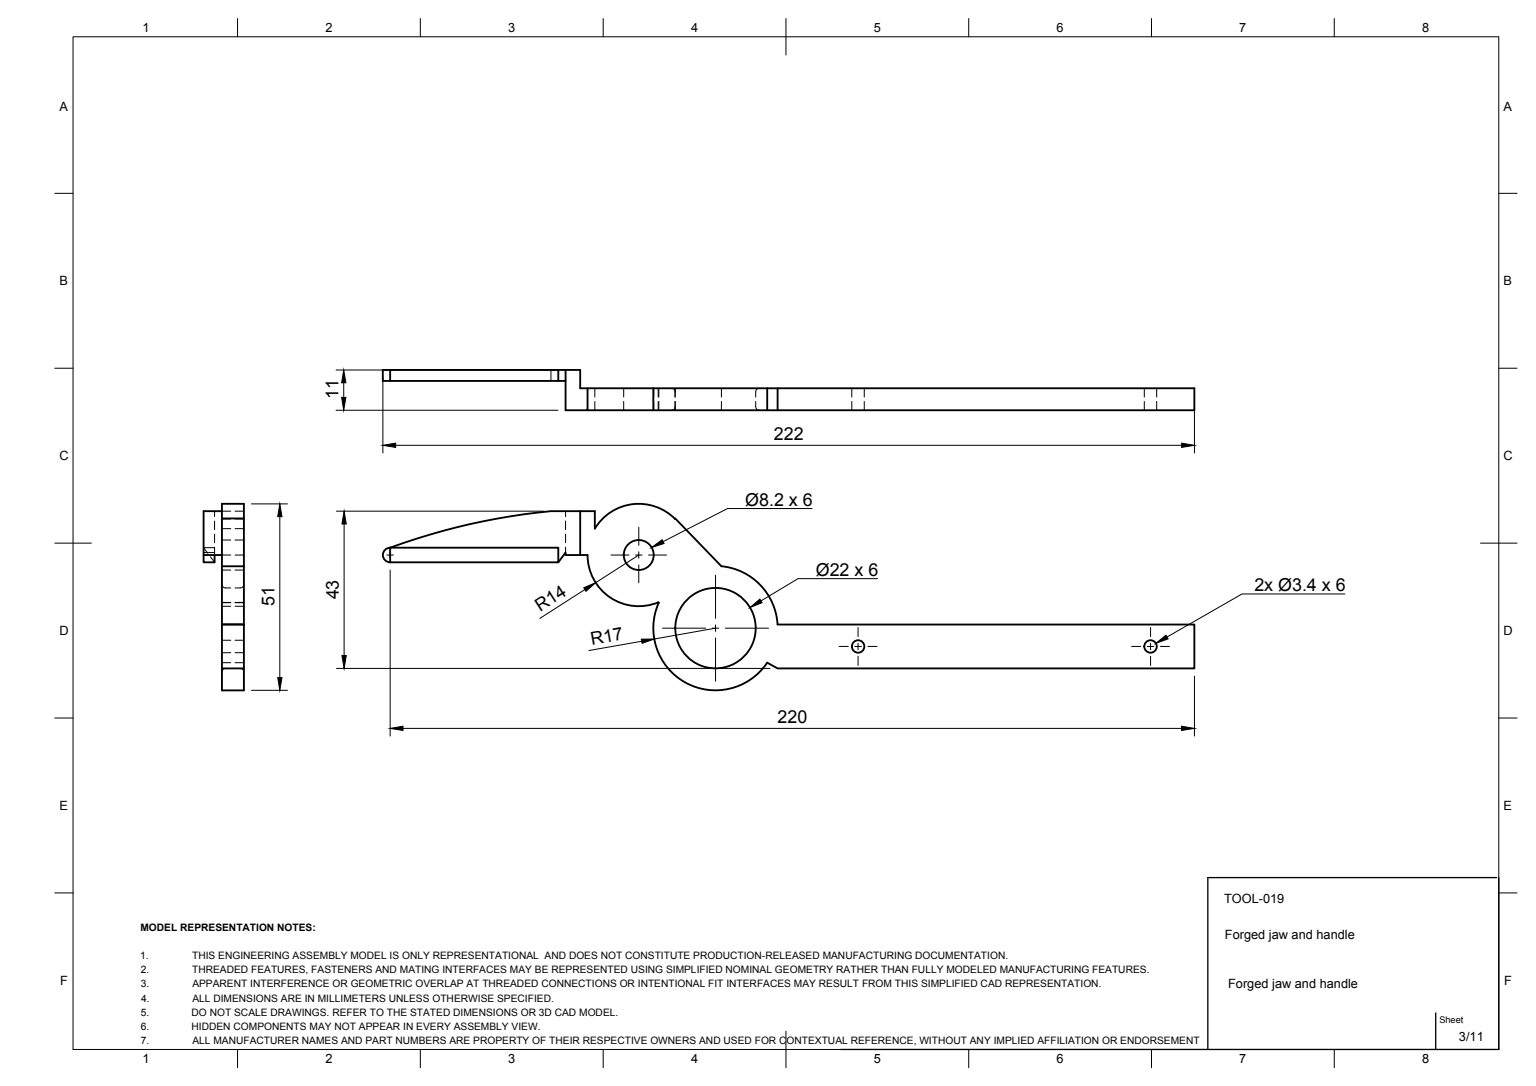
ISO-10303-21;
HEADER;
/* Generated by software containing ST-Developer
 * from STEP Tools, Inc. (www.steptools.com) 
 */

FILE_DESCRIPTION(
/* description */ (''),
/* implementation_level */ '2;1');

FILE_NAME(
/* name */ 'Forged jaw and handle.step',
/* time_stamp */ '2026-11-10T09:14:46-08:00',
/* author */ (''),
/* organization */ (''),
/* preprocessor_version */ 'ST-DEVELOPER v20.2',
/* originating_system */ 'Autodesk Translation Framework v15.17.0.0',
/* authorisation */ '');

FILE_SCHEMA (('AUTOMOTIVE_DESIGN { 1 0 10303 214 3 1 1 }'));
ENDSEC;

DATA;
#10=MECHANICAL_DESIGN_GEOMETRIC_PRESENTATION_REPRESENTATION('',(#558),#19471);
#538=SHAPE_REPRESENTATION_RELATIONSHIP('SRR','None',#19517,#548);
#548=ADVANCED_BREP_SHAPE_REPRESENTATION('',(#568),#19460);
#558=STYLED_ITEM('',(#19581),#568);
#568=MANIFOLD_SOLID_BREP('Body1',#7151);
#578=TOROIDAL_SURFACE('',#7315,1.2,0.1);
#579=TOROIDAL_SURFACE('',#7321,1.2,0.1);
#582=FACE_BOUND('',#1246,.T.);
#583=FACE_BOUND('',#1247,.T.);
#584=FACE_BOUND('',#1248,.T.);
#585=FACE_BOUND('',#1249,.T.);
#586=FACE_BOUND('',#1254,.T.);
#587=FACE_BOUND('',#1255,.T.);
#588=FACE_BOUND('',#1256,.T.);
#589=FACE_BOUND('',#1257,.T.);
#653=PLANE('',#7283);
#654=PLANE('',#7284);
#655=PLANE('',#7285);
#656=PLANE('',#7286);
#657=PLANE('',#7288);
#658=PLANE('',#7294);
#659=PLANE('',#7295);
#660=PLANE('',#7296);
#661=PLANE('',#7297);
#662=PLANE('',#7298);
#663=PLANE('',#7299);
#664=PLANE('',#7300);
#665=PLANE('',#7306);
#666=PLANE('',#7311);
#667=PLANE('',#7325);
#668=PLANE('',#7326);
#669=PLANE('',#7327);
#670=PLANE('',#7328);
#671=PLANE('',#7329);
#672=PLANE('',#7330);
#673=PLANE('',#7331);
#674=PLANE('',#7332);
#820=FACE_OUTER_BOUND('',#1229,.T.);
#821=FACE_OUTER_BOUND('',#1230,.T.);
#822=FACE_OUTER_BOUND('',#1231,.T.);
#823=FACE_OUTER_BOUND('',#1232,.T.);
#824=FACE_OUTER_BOUND('',#1233,.T.);
#825=FACE_OUTER_BOUND('',#1234,.T.);
#826=FACE_OUTER_BOUND('',#1235,.T.);
#827=FACE_OUTER_BOUND('',#1236,.T.);
#828=FACE_OUTER_BOUND('',#1237,.T.);
#829=FACE_OUTER_BOUND('',#1238,.T.);
#830=FACE_OUTER_BOUND('',#1239,.T.);
#831=FACE_OUTER_BOUND('',#1240,.T.);
#832=FACE_OUTER_BOUND('',#1241,.T.);
#833=FACE_OUTER_BOUND('',#1242,.T.);
#834=FACE_OUTER_BOUND('',#1243,.T.);
#835=FACE_OUTER_BOUND('',#1244,.T.);
#836=FACE_OUTER_BOUND('',#1245,.T.);
#837=FACE_OUTER_BOUND('',#1250,.T.);
#838=FACE_OUTER_BOUND('',#1251,.T.);
#839=FACE_OUTER_BOUND('',#1252,.T.);
#840=FACE_OUTER_BOUND('',#1253,.T.);
#841=FACE_OUTER_BOUND('',#1258,.T.);
#842=FACE_OUTER_BOUND('',#1259,.T.);
#843=FACE_OUTER_BOUND('',#1260,.T.);
#844=FACE_OUTER_BOUND('',#1261,.T.);
#845=FACE_OUTER_BOUND('',#1262,.T.);
#846=FACE_OUTER_BOUND('',#1263,.T.);
#847=FACE_OUTER_BOUND('',#1264,.T.);
#848=FACE_OUTER_BOUND('',#1265,.T.);
#849=FACE_OUTER_BOUND('',#1266,.T.);
#850=FACE_OUTER_BOUND('',#1267,.T.);
#851=FACE_OUTER_BOUND('',#1268,.T.);
#852=FACE_OUTER_BOUND('',#1269,.T.);
#853=FACE_OUTER_BOUND('',#1270,.T.);
#1229=EDGE_LOOP('',(#4541,#4542,#4543,#4544));
#1230=EDGE_LOOP('',(#4545,#4546,#4547,#4548));
#1231=EDGE_LOOP('',(#4549,#4550,#4551,#4552));
#1232=EDGE_LOOP('',(#4553,#4554,#4555));
#1233=EDGE_LOOP('',(#4556,#4557,#4558,#4559));
#1234=EDGE_LOOP('',(#4560,#4561,#4562));
#1235=EDGE_LOOP('',(#4563,#4564,#4565,#4566,#4567,#4568,#4569,#4570));
#1236=EDGE_LOOP('',(#4571,#4572,#4573,#4574));
#1237=EDGE_LOOP('',(#4575,#4576,#4577,#4578));
#1238=EDGE_LOOP('',(#4579,#4580,#4581,#4582));
#1239=EDGE_LOOP('',(#4583,#4584,#4585,#4586,#4587,#4588));
#1240=EDGE_LOOP('',(#4589,#4590,#4591,#4592,#4593,#4594));
#1241=EDGE_LOOP('',(#4595,#4596,#4597,#4598,#4599,#4600,#4601,#4602));
#1242=EDGE_LOOP('',(#4603,#4604,#4605,#4606));
#1243=EDGE_LOOP('',(#4607,#4608));
#1244=EDGE_LOOP('',(#4609,#4610,#4611,#4612,#4613,#4614));
#1245=EDGE_LOOP('',(#4615,#4616,#4617,#4618,#4619,#4620,#4621,#4622,#4623,
#4624,#4625,#4626,#4627,#4628,#4629,#4630));
#1246=EDGE_LOOP('',(#4631));
#1247=EDGE_LOOP('',(#4632));
#1248=EDGE_LOOP('',(#4633));
#1249=EDGE_LOOP('',(#4634));
#1250=EDGE_LOOP('',(#4635,#4636,#4637,#4638));
#1251=EDGE_LOOP('',(#4639,#4640,#4641,#4642));
#1252=EDGE_LOOP('',(#4643,#4644,#4645,#4646));
#1253=EDGE_LOOP('',(#4647,#4648,#4649,#4650,#4651,#4652,#4653,#4654,#4655,
#4656,#4657,#4658,#4659,#4660,#4661,#4662));
#1254=EDGE_LOOP('',(#4663));
#1255=EDGE_LOOP('',(#4664));
#1256=EDGE_LOOP('',(#4665));
#1257=EDGE_LOOP('',(#4666));
#1258=EDGE_LOOP('',(#4667,#4668,#4669,#4670));
#1259=EDGE_LOOP('',(#4671,#4672,#4673,#4674,#4675));
#1260=EDGE_LOOP('',(#4676,#4677,#4678,#4679,#4680));
#1261=EDGE_LOOP('',(#4681,#4682,#4683,#4684));
#1262=EDGE_LOOP('',(#4685,#4686,#4687,#4688));
#1263=EDGE_LOOP('',(#4689,#4690,#4691,#4692));
#1264=EDGE_LOOP('',(#4693,#4694,#4695,#4696));
#1265=EDGE_LOOP('',(#4697,#4698,#4699,#4700));
#1266=EDGE_LOOP('',(#4701,#4702,#4703,#4704));
#1267=EDGE_LOOP('',(#4705,#4706,#4707,#4708));
#1268=EDGE_LOOP('',(#4709,#4710,#4711,#4712));
#1269=EDGE_LOOP('',(#4713,#4714,#4715,#4716));
#1270=EDGE_LOOP('',(#4717,#4718,#4719,#4720));
#1709=LINE('',#9393,#2183);
#1710=LINE('',#9399,#2184);
#1711=LINE('',#9405,#2185);
#1712=LINE('',#9410,#2186);
#1713=LINE('',#9412,#2187);
#1714=LINE('',#9413,#2188);
#1715=LINE('',#9417,#2189);
#1716=LINE('',#9418,#2190);
#1717=LINE('',#9419,#2191);
#1718=LINE('',#9422,#2192);
#1719=LINE('',#9423,#2193);
#1720=LINE('',#9426,#2194);
#1721=LINE('',#9428,#2195);
#1722=LINE('',#9430,#2196);
#1723=LINE('',#9432,#2197);
#1724=LINE('',#9434,#2198);
#1725=LINE('',#9438,#2199);
#1726=LINE('',#9439,#2200);
#1727=LINE('',#9444,#2201);
#1728=LINE('',#9448,#2202);
#1729=LINE('',#9451,#2203);
#1730=LINE('',#9452,#2204);
#1731=LINE('',#9455,#2205);
#1732=LINE('',#9457,#2206);
#1733=LINE('',#9458,#2207);
#1734=LINE('',#9461,#2208);
#1735=LINE('',#9463,#2209);
#1736=LINE('',#9465,#2210);
#1737=LINE('',#9466,#2211);
#1738=LINE('',#9469,#2212);
#1739=LINE('',#9470,#2213);
#1740=LINE('',#9474,#2214);
#1741=LINE('',#9476,#2215);
#1742=LINE('',#9477,#2216);
#1743=LINE('',#9480,#2217);
#1744=LINE('',#9484,#2218);
#1745=LINE('',#9486,#2219);
#1746=LINE('',#9490,#2220);
#1747=LINE('',#9492,#2221);
#1748=LINE('',#9494,#2222);
#1749=LINE('',#9496,#2223);
#1750=LINE('',#9498,#2224);
#1751=LINE('',#9502,#2225);
#1752=LINE('',#9508,#2226);
#1753=LINE('',#9509,#2227);
#1754=LINE('',#9512,#2228);
#1755=LINE('',#9517,#2229);
#1756=LINE('',#9520,#2230);
#1757=LINE('',#9524,#2231);
#1758=LINE('',#9526,#2232);
#1759=LINE('',#9528,#2233);
#1760=LINE('',#9530,#2234);
#1761=LINE('',#9532,#2235);
#1762=LINE('',#9536,#2236);
#1763=LINE('',#9537,#2237);
#1764=LINE('',#9549,#2238);
#1765=LINE('',#9553,#2239);
#1766=LINE('',#9554,#2240);
#1767=LINE('',#9556,#2241);
#1768=LINE('',#9557,#2242);
#1769=LINE('',#9559,#2243);
#1770=LINE('',#9561,#2244);
#1771=LINE('',#9564,#2245);
#1772=LINE('',#9567,#2246);
#1773=LINE('',#9569,#2247);
#2183=VECTOR('',#7827,0.17);
#2184=VECTOR('',#7834,0.17);
#2185=VECTOR('',#7841,0.41);
#2186=VECTOR('',#7846,1.);
#2187=VECTOR('',#7847,1.);
#2188=VECTOR('',#7848,1.);
#2189=VECTOR('',#7851,1.);
#2190=VECTOR('',#7852,1.);
#2191=VECTOR('',#7853,1.);
#2192=VECTOR('',#7856,1.);
#2193=VECTOR('',#7857,1.);
#2194=VECTOR('',#7860,1.);
#2195=VECTOR('',#7861,1.);
#2196=VECTOR('',#7862,1.);
#2197=VECTOR('',#7863,1.);
#2198=VECTOR('',#7864,1.);
#2199=VECTOR('',#7869,1.);
#2200=VECTOR('',#7870,1.);
#2201=VECTOR('',#7877,1.);
#2202=VECTOR('',#7882,1.);
#2203=VECTOR('',#7885,1.);
#2204=VECTOR('',#7886,1.);
#2205=VECTOR('',#7889,1.);
#2206=VECTOR('',#7890,1.);
#2207=VECTOR('',#7891,1.);
#2208=VECTOR('',#7894,1.);
#2209=VECTOR('',#7895,1.);
#2210=VECTOR('',#7896,1.);
#2211=VECTOR('',#7897,1.);
#2212=VECTOR('',#7900,1.);
#2213=VECTOR('',#7901,1.);
#2214=VECTOR('',#7906,1.);
#2215=VECTOR('',#7907,1.);
#2216=VECTOR('',#7908,1.);
#2217=VECTOR('',#7911,1.);
#2218=VECTOR('',#7914,1.);
#2219=VECTOR('',#7915,1.);
#2220=VECTOR('',#7918,1.);
#2221=VECTOR('',#7919,1.);
#2222=VECTOR('',#7920,1.);
#2223=VECTOR('',#7921,1.);
#2224=VECTOR('',#7922,1.);
#2225=VECTOR('',#7925,1.);
#2226=VECTOR('',#7932,1.);
#2227=VECTOR('',#7933,1.);
#2228=VECTOR('',#7936,1.);
#2229=VECTOR('',#7943,1.);
#2230=VECTOR('',#7946,1.);
#2231=VECTOR('',#7949,1.);
#2232=VECTOR('',#7950,1.);
#2233=VECTOR('',#7951,1.);
#2234=VECTOR('',#7952,1.);
#2235=VECTOR('',#7953,1.);
#2236=VECTOR('',#7956,1.);
#2237=VECTOR('',#7957,1.);
#2238=VECTOR('',#7972,1.1);
#2239=VECTOR('',#7979,1.);
#2240=VECTOR('',#7980,1.);
#2241=VECTOR('',#7983,1.);
#2242=VECTOR('',#7984,1.);
#2243=VECTOR('',#7987,1.);
#2244=VECTOR('',#7990,1.);
#2245=VECTOR('',#7995,1.);
#2246=VECTOR('',#8000,1.);
#2247=VECTOR('',#8003,1.);
#2657=CIRCLE('',#7275,0.17);
#2658=CIRCLE('',#7276,0.17);
#2659=CIRCLE('',#7278,0.17);
#2660=CIRCLE('',#7279,0.17);
#2661=CIRCLE('',#7281,0.41);
#2662=CIRCLE('',#7282,0.41);
#2663=CIRCLE('',#7287,17.7082646568653);
#2664=CIRCLE('',#7290,0.2);
#2665=CIRCLE('',#7291,0.2);
#2666=CIRCLE('',#7293,17.7082646568653);
#2667=CIRCLE('',#7301,1.4);
#2668=CIRCLE('',#7302,1.7);
#2669=CIRCLE('',#7303,1.7);
#2670=CIRCLE('',#7304,1.4);
#2671=CIRCLE('',#7305,1.2);
#2672=CIRCLE('',#7308,1.4);
#2673=CIRCLE('',#7310,1.4);
#2674=CIRCLE('',#7312,1.7);
#2675=CIRCLE('',#7313,1.7);
#2676=CIRCLE('',#7314,1.2);
#2677=CIRCLE('',#7316,0.1);
#2678=CIRCLE('',#7317,1.1);
#2679=CIRCLE('',#7319,1.1);
#2680=CIRCLE('',#7320,1.1);
#2681=CIRCLE('',#7322,0.1);
#2847=VERTEX_POINT('',#9390);
#2848=VERTEX_POINT('',#9392);
#2849=VERTEX_POINT('',#9396);
#2850=VERTEX_POINT('',#9398);
#2851=VERTEX_POINT('',#9402);
#2852=VERTEX_POINT('',#9404);
#2853=VERTEX_POINT('',#9408);
#2854=VERTEX_POINT('',#9409);
#2855=VERTEX_POINT('',#9411);
#2856=VERTEX_POINT('',#9415);
#2857=VERTEX_POINT('',#9416);
#2858=VERTEX_POINT('',#9421);
#2859=VERTEX_POINT('',#9425);
#2860=VERTEX_POINT('',#9427);
#2861=VERTEX_POINT('',#9429);
#2862=VERTEX_POINT('',#9431);
#2863=VERTEX_POINT('',#9433);
#2864=VERTEX_POINT('',#9437);
#2865=VERTEX_POINT('',#9441);
#2866=VERTEX_POINT('',#9446);
#2867=VERTEX_POINT('',#9450);
#2868=VERTEX_POINT('',#9454);
#2869=VERTEX_POINT('',#9456);
#2870=VERTEX_POINT('',#9460);
#2871=VERTEX_POINT('',#9462);
#2872=VERTEX_POINT('',#9464);
#2873=VERTEX_POINT('',#9468);
#2874=VERTEX_POINT('',#9473);
#2875=VERTEX_POINT('',#9475);
#2876=VERTEX_POINT('',#9479);
#2877=VERTEX_POINT('',#9481);
#2878=VERTEX_POINT('',#9483);
#2879=VERTEX_POINT('',#9485);
#2880=VERTEX_POINT('',#9487);
#2881=VERTEX_POINT('',#9489);
#2882=VERTEX_POINT('',#9491);
#2883=VERTEX_POINT('',#9493);
#2884=VERTEX_POINT('',#9495);
#2885=VERTEX_POINT('',#9497);
#2886=VERTEX_POINT('',#9499);
#2887=VERTEX_POINT('',#9501);
#2888=VERTEX_POINT('',#9504);
#2889=VERTEX_POINT('',#9507);
#2890=VERTEX_POINT('',#9511);
#2891=VERTEX_POINT('',#9515);
#2892=VERTEX_POINT('',#9519);
#2893=VERTEX_POINT('',#9521);
#2894=VERTEX_POINT('',#9523);
#2895=VERTEX_POINT('',#9525);
#2896=VERTEX_POINT('',#9527);
#2897=VERTEX_POINT('',#9529);
#2898=VERTEX_POINT('',#9531);
#2899=VERTEX_POINT('',#9533);
#2900=VERTEX_POINT('',#9535);
#2901=VERTEX_POINT('',#9538);
#2902=VERTEX_POINT('',#9541);
#2903=VERTEX_POINT('',#9545);
#2904=VERTEX_POINT('',#9546);
#3511=EDGE_CURVE('',#2847,#2847,#2657,.T.);
#3512=EDGE_CURVE('',#2847,#2848,#1709,.T.);
#3513=EDGE_CURVE('',#2848,#2848,#2658,.T.);
#3514=EDGE_CURVE('',#2849,#2849,#2659,.T.);
#3515=EDGE_CURVE('',#2849,#2850,#1710,.T.);
#3516=EDGE_CURVE('',#2850,#2850,#2660,.T.);
#3517=EDGE_CURVE('',#2851,#2851,#2661,.T.);
#3518=EDGE_CURVE('',#2851,#2852,#1711,.T.);
#3519=EDGE_CURVE('',#2852,#2852,#2662,.T.);
#3520=EDGE_CURVE('',#2853,#2854,#1712,.T.);
#3521=EDGE_CURVE('',#2855,#2853,#1713,.T.);
#3522=EDGE_CURVE('',#2855,#2854,#1714,.T.);
#3523=EDGE_CURVE('',#2856,#2857,#1715,.T.);
#3524=EDGE_CURVE('',#2855,#2856,#1716,.T.);
#3525=EDGE_CURVE('',#2857,#2853,#1717,.T.);
#3526=EDGE_CURVE('',#2858,#2857,#1718,.T.);
#3527=EDGE_CURVE('',#2856,#2858,#1719,.T.);
#3528=EDGE_CURVE('',#2854,#2859,#1720,.T.);
#3529=EDGE_CURVE('',#2859,#2860,#1721,.T.);
#3530=EDGE_CURVE('',#2860,#2861,#1722,.T.);
#3531=EDGE_CURVE('',#2861,#2862,#1723,.T.);
#3532=EDGE_CURVE('',#2862,#2863,#1724,.T.);
#3533=EDGE_CURVE('',#2863,#2857,#2663,.T.);
#3534=EDGE_CURVE('',#2859,#2864,#1725,.T.);
#3535=EDGE_CURVE('',#2864,#2855,#1726,.T.);
#3536=EDGE_CURVE('',#2865,#2856,#2664,.T.);
#3537=EDGE_CURVE('',#2857,#2858,#2665,.T.);
#3538=EDGE_CURVE('',#2865,#2857,#1727,.T.);
#3539=EDGE_CURVE('',#2866,#2865,#2666,.T.);
#3540=EDGE_CURVE('',#2866,#2863,#1728,.T.);
#3541=EDGE_CURVE('',#2864,#2867,#1729,.T.);
#3542=EDGE_CURVE('',#2866,#2867,#1730,.T.);
#3543=EDGE_CURVE('',#2868,#2867,#1731,.T.);
#3544=EDGE_CURVE('',#2869,#2868,#1732,.T.);
#3545=EDGE_CURVE('',#2869,#2860,#1733,.T.);
#3546=EDGE_CURVE('',#2870,#2862,#1734,.T.);
#3547=EDGE_CURVE('',#2871,#2870,#1735,.T.);
#3548=EDGE_CURVE('',#2872,#2871,#1736,.T.);
#3549=EDGE_CURVE('',#2868,#2872,#1737,.T.);
#3550=EDGE_CURVE('',#2873,#2861,#1738,.T.);
#3551=EDGE_CURVE('',#2870,#2873,#1739,.T.);
#3552=EDGE_CURVE('',#2874,#2869,#1740,.T.);
#3553=EDGE_CURVE('',#2875,#2874,#1741,.T.);
#3554=EDGE_CURVE('',#2873,#2875,#1742,.T.);
#3555=EDGE_CURVE('',#2872,#2876,#1743,.T.);
#3556=EDGE_CURVE('',#2877,#2876,#2667,.T.);
#3557=EDGE_CURVE('',#2878,#2877,#1744,.T.);
#3558=EDGE_CURVE('',#2879,#2878,#1745,.T.);
#3559=EDGE_CURVE('',#2880,#2879,#2668,.T.);
#3560=EDGE_CURVE('',#2881,#2880,#1746,.T.);
#3561=EDGE_CURVE('',#2882,#2881,#1747,.T.);
#3562=EDGE_CURVE('',#2883,#2882,#1748,.T.);
#3563=EDGE_CURVE('',#2884,#2883,#1749,.T.);
#3564=EDGE_CURVE('',#2885,#2884,#1750,.T.);
#3565=EDGE_CURVE('',#2886,#2885,#2669,.T.);
#3566=EDGE_CURVE('',#2887,#2886,#1751,.T.);
#3567=EDGE_CURVE('',#2874,#2887,#2670,.T.);
#3568=EDGE_CURVE('',#2888,#2888,#2671,.T.);
#3569=EDGE_CURVE('',#2876,#2889,#1752,.T.);
#3570=EDGE_CURVE('',#2889,#2871,#1753,.T.);
#3571=EDGE_CURVE('',#2887,#2890,#1754,.T.);
#3572=EDGE_CURVE('',#2875,#2890,#2672,.T.);
#3573=EDGE_CURVE('',#2891,#2889,#2673,.T.);
#3574=EDGE_CURVE('',#2891,#2877,#1755,.T.);
#3575=EDGE_CURVE('',#2890,#2892,#1756,.T.);
#3576=EDGE_CURVE('',#2892,#2893,#2674,.T.);
#3577=EDGE_CURVE('',#2893,#2894,#1757,.T.);
#3578=EDGE_CURVE('',#2894,#2895,#1758,.T.);
#3579=EDGE_CURVE('',#2895,#2896,#1759,.T.);
#3580=EDGE_CURVE('',#2896,#2897,#1760,.T.);
#3581=EDGE_CURVE('',#2897,#2898,#1761,.T.);
#3582=EDGE_CURVE('',#2898,#2899,#2675,.T.);
#3583=EDGE_CURVE('',#2899,#2900,#1762,.T.);
#3584=EDGE_CURVE('',#2900,#2891,#1763,.T.);
#3585=EDGE_CURVE('',#2901,#2901,#2676,.T.);
#3586=EDGE_CURVE('',#2888,#2902,#2677,.T.);
#3587=EDGE_CURVE('',#2902,#2902,#2678,.T.);
#3588=EDGE_CURVE('',#2903,#2904,#2679,.T.);
#3589=EDGE_CURVE('',#2904,#2903,#2680,.T.);
#3590=EDGE_CURVE('',#2904,#2902,#1764,.T.);
#3591=EDGE_CURVE('',#2901,#2903,#2681,.T.);
#3592=EDGE_CURVE('',#2899,#2879,#1765,.T.);
#3593=EDGE_CURVE('',#2880,#2898,#1766,.T.);
#3594=EDGE_CURVE('',#2886,#2892,#1767,.T.);
#3595=EDGE_CURVE('',#2893,#2885,#1768,.T.);
#3596=EDGE_CURVE('',#2884,#2894,#1769,.T.);
#3597=EDGE_CURVE('',#2881,#2897,#1770,.T.);
#3598=EDGE_CURVE('',#2878,#2900,#1771,.T.);
#3599=EDGE_CURVE('',#2882,#2896,#1772,.T.);
#3600=EDGE_CURVE('',#2883,#2895,#1773,.T.);
#4541=ORIENTED_EDGE('',*,*,#3511,.F.);
#4542=ORIENTED_EDGE('',*,*,#3512,.T.);
#4543=ORIENTED_EDGE('',*,*,#3513,.F.);
#4544=ORIENTED_EDGE('',*,*,#3512,.F.);
#4545=ORIENTED_EDGE('',*,*,#3514,.F.);
#4546=ORIENTED_EDGE('',*,*,#3515,.T.);
#4547=ORIENTED_EDGE('',*,*,#3516,.F.);
#4548=ORIENTED_EDGE('',*,*,#3515,.F.);
#4549=ORIENTED_EDGE('',*,*,#3517,.F.);
#4550=ORIENTED_EDGE('',*,*,#3518,.T.);
#4551=ORIENTED_EDGE('',*,*,#3519,.F.);
#4552=ORIENTED_EDGE('',*,*,#3518,.F.);
#4553=ORIENTED_EDGE('',*,*,#3520,.F.);
#4554=ORIENTED_EDGE('',*,*,#3521,.F.);
#4555=ORIENTED_EDGE('',*,*,#3522,.T.);
#4556=ORIENTED_EDGE('',*,*,#3523,.F.);
#4557=ORIENTED_EDGE('',*,*,#3524,.F.);
#4558=ORIENTED_EDGE('',*,*,#3521,.T.);
#4559=ORIENTED_EDGE('',*,*,#3525,.F.);
#4560=ORIENTED_EDGE('',*,*,#3526,.F.);
#4561=ORIENTED_EDGE('',*,*,#3527,.F.);
#4562=ORIENTED_EDGE('',*,*,#3523,.T.);
#4563=ORIENTED_EDGE('',*,*,#3525,.T.);
#4564=ORIENTED_EDGE('',*,*,#3520,.T.);
#4565=ORIENTED_EDGE('',*,*,#3528,.T.);
#4566=ORIENTED_EDGE('',*,*,#3529,.T.);
#4567=ORIENTED_EDGE('',*,*,#3530,.T.);
#4568=ORIENTED_EDGE('',*,*,#3531,.T.);
#4569=ORIENTED_EDGE('',*,*,#3532,.T.);
#4570=ORIENTED_EDGE('',*,*,#3533,.T.);
#4571=ORIENTED_EDGE('',*,*,#3534,.F.);
#4572=ORIENTED_EDGE('',*,*,#3528,.F.);
#4573=ORIENTED_EDGE('',*,*,#3522,.F.);
#4574=ORIENTED_EDGE('',*,*,#3535,.F.);
#4575=ORIENTED_EDGE('',*,*,#3536,.T.);
#4576=ORIENTED_EDGE('',*,*,#3527,.T.);
#4577=ORIENTED_EDGE('',*,*,#3537,.F.);
#4578=ORIENTED_EDGE('',*,*,#3538,.F.);
#4579=ORIENTED_EDGE('',*,*,#3539,.T.);
#4580=ORIENTED_EDGE('',*,*,#3538,.T.);
#4581=ORIENTED_EDGE('',*,*,#3533,.F.);
#4582=ORIENTED_EDGE('',*,*,#3540,.F.);
#4583=ORIENTED_EDGE('',*,*,#3541,.F.);
#4584=ORIENTED_EDGE('',*,*,#3535,.T.);
#4585=ORIENTED_EDGE('',*,*,#3524,.T.);
#4586=ORIENTED_EDGE('',*,*,#3536,.F.);
#4587=ORIENTED_EDGE('',*,*,#3539,.F.);
#4588=ORIENTED_EDGE('',*,*,#3542,.T.);
#4589=ORIENTED_EDGE('',*,*,#3534,.T.);
#4590=ORIENTED_EDGE('',*,*,#3541,.T.);
#4591=ORIENTED_EDGE('',*,*,#3543,.F.);
#4592=ORIENTED_EDGE('',*,*,#3544,.F.);
#4593=ORIENTED_EDGE('',*,*,#3545,.T.);
#4594=ORIENTED_EDGE('',*,*,#3529,.F.);
#4595=ORIENTED_EDGE('',*,*,#3546,.F.);
#4596=ORIENTED_EDGE('',*,*,#3547,.F.);
#4597=ORIENTED_EDGE('',*,*,#3548,.F.);
#4598=ORIENTED_EDGE('',*,*,#3549,.F.);
#4599=ORIENTED_EDGE('',*,*,#3543,.T.);
#4600=ORIENTED_EDGE('',*,*,#3542,.F.);
#4601=ORIENTED_EDGE('',*,*,#3540,.T.);
#4602=ORIENTED_EDGE('',*,*,#3532,.F.);
#4603=ORIENTED_EDGE('',*,*,#3531,.F.);
#4604=ORIENTED_EDGE('',*,*,#3550,.F.);
#4605=ORIENTED_EDGE('',*,*,#3551,.F.);
#4606=ORIENTED_EDGE('',*,*,#3546,.T.);
#4607=ORIENTED_EDGE('',*,*,#3526,.T.);
#4608=ORIENTED_EDGE('',*,*,#3537,.T.);
#4609=ORIENTED_EDGE('',*,*,#3552,.F.);
#4610=ORIENTED_EDGE('',*,*,#3553,.F.);
#4611=ORIENTED_EDGE('',*,*,#3554,.F.);
#4612=ORIENTED_EDGE('',*,*,#3550,.T.);
#4613=ORIENTED_EDGE('',*,*,#3530,.F.);
#4614=ORIENTED_EDGE('',*,*,#3545,.F.);
#4615=ORIENTED_EDGE('',*,*,#3549,.T.);
#4616=ORIENTED_EDGE('',*,*,#3555,.T.);
#4617=ORIENTED_EDGE('',*,*,#3556,.F.);
#4618=ORIENTED_EDGE('',*,*,#3557,.F.);
#4619=ORIENTED_EDGE('',*,*,#3558,.F.);
#4620=ORIENTED_EDGE('',*,*,#3559,.F.);
#4621=ORIENTED_EDGE('',*,*,#3560,.F.);
#4622=ORIENTED_EDGE('',*,*,#3561,.F.);
#4623=ORIENTED_EDGE('',*,*,#3562,.F.);
#4624=ORIENTED_EDGE('',*,*,#3563,.F.);
#4625=ORIENTED_EDGE('',*,*,#3564,.F.);
#4626=ORIENTED_EDGE('',*,*,#3565,.F.);
#4627=ORIENTED_EDGE('',*,*,#3566,.F.);
#4628=ORIENTED_EDGE('',*,*,#3567,.F.);
#4629=ORIENTED_EDGE('',*,*,#3552,.T.);
#4630=ORIENTED_EDGE('',*,*,#3544,.T.);
#4631=ORIENTED_EDGE('',*,*,#3513,.T.);
#4632=ORIENTED_EDGE('',*,*,#3516,.T.);
#4633=ORIENTED_EDGE('',*,*,#3519,.T.);
#4634=ORIENTED_EDGE('',*,*,#3568,.F.);
#4635=ORIENTED_EDGE('',*,*,#3569,.F.);
#4636=ORIENTED_EDGE('',*,*,#3555,.F.);
#4637=ORIENTED_EDGE('',*,*,#3548,.T.);
#4638=ORIENTED_EDGE('',*,*,#3570,.F.);
#4639=ORIENTED_EDGE('',*,*,#3553,.T.);
#4640=ORIENTED_EDGE('',*,*,#3567,.T.);
#4641=ORIENTED_EDGE('',*,*,#3571,.T.);
#4642=ORIENTED_EDGE('',*,*,#3572,.F.);
#4643=ORIENTED_EDGE('',*,*,#3569,.T.);
#4644=ORIENTED_EDGE('',*,*,#3573,.F.);
#4645=ORIENTED_EDGE('',*,*,#3574,.T.);
#4646=ORIENTED_EDGE('',*,*,#3556,.T.);
#4647=ORIENTED_EDGE('',*,*,#3551,.T.);
#4648=ORIENTED_EDGE('',*,*,#3554,.T.);
#4649=ORIENTED_EDGE('',*,*,#3572,.T.);
#4650=ORIENTED_EDGE('',*,*,#3575,.T.);
#4651=ORIENTED_EDGE('',*,*,#3576,.T.);
#4652=ORIENTED_EDGE('',*,*,#3577,.T.);
#4653=ORIENTED_EDGE('',*,*,#3578,.T.);
#4654=ORIENTED_EDGE('',*,*,#3579,.T.);
#4655=ORIENTED_EDGE('',*,*,#3580,.T.);
#4656=ORIENTED_EDGE('',*,*,#3581,.T.);
#4657=ORIENTED_EDGE('',*,*,#3582,.T.);
#4658=ORIENTED_EDGE('',*,*,#3583,.T.);
#4659=ORIENTED_EDGE('',*,*,#3584,.T.);
#4660=ORIENTED_EDGE('',*,*,#3573,.T.);
#4661=ORIENTED_EDGE('',*,*,#3570,.T.);
#4662=ORIENTED_EDGE('',*,*,#3547,.T.);
#4663=ORIENTED_EDGE('',*,*,#3511,.T.);
#4664=ORIENTED_EDGE('',*,*,#3514,.T.);
#4665=ORIENTED_EDGE('',*,*,#3517,.T.);
#4666=ORIENTED_EDGE('',*,*,#3585,.F.);
#4667=ORIENTED_EDGE('',*,*,#3568,.T.);
#4668=ORIENTED_EDGE('',*,*,#3586,.T.);
#4669=ORIENTED_EDGE('',*,*,#3587,.T.);
#4670=ORIENTED_EDGE('',*,*,#3586,.F.);
#4671=ORIENTED_EDGE('',*,*,#3588,.F.);
#4672=ORIENTED_EDGE('',*,*,#3589,.F.);
#4673=ORIENTED_EDGE('',*,*,#3590,.T.);
#4674=ORIENTED_EDGE('',*,*,#3587,.F.);
#4675=ORIENTED_EDGE('',*,*,#3590,.F.);
#4676=ORIENTED_EDGE('',*,*,#3585,.T.);
#4677=ORIENTED_EDGE('',*,*,#3591,.T.);
#4678=ORIENTED_EDGE('',*,*,#3588,.T.);
#4679=ORIENTED_EDGE('',*,*,#3589,.T.);
#4680=ORIENTED_EDGE('',*,*,#3591,.F.);
#4681=ORIENTED_EDGE('',*,*,#3592,.F.);
#4682=ORIENTED_EDGE('',*,*,#3582,.F.);
#4683=ORIENTED_EDGE('',*,*,#3593,.F.);
#4684=ORIENTED_EDGE('',*,*,#3559,.T.);
#4685=ORIENTED_EDGE('',*,*,#3594,.F.);
#4686=ORIENTED_EDGE('',*,*,#3565,.T.);
#4687=ORIENTED_EDGE('',*,*,#3595,.F.);
#4688=ORIENTED_EDGE('',*,*,#3576,.F.);
#4689=ORIENTED_EDGE('',*,*,#3595,.T.);
#4690=ORIENTED_EDGE('',*,*,#3564,.T.);
#4691=ORIENTED_EDGE('',*,*,#3596,.T.);
#4692=ORIENTED_EDGE('',*,*,#3577,.F.);
#4693=ORIENTED_EDGE('',*,*,#3593,.T.);
#4694=ORIENTED_EDGE('',*,*,#3581,.F.);
#4695=ORIENTED_EDGE('',*,*,#3597,.F.);
#4696=ORIENTED_EDGE('',*,*,#3560,.T.);
#4697=ORIENTED_EDGE('',*,*,#3594,.T.);
#4698=ORIENTED_EDGE('',*,*,#3575,.F.);
#4699=ORIENTED_EDGE('',*,*,#3571,.F.);
#4700=ORIENTED_EDGE('',*,*,#3566,.T.);
#4701=ORIENTED_EDGE('',*,*,#3574,.F.);
#4702=ORIENTED_EDGE('',*,*,#3584,.F.);
#4703=ORIENTED_EDGE('',*,*,#3598,.F.);
#4704=ORIENTED_EDGE('',*,*,#3557,.T.);
#4705=ORIENTED_EDGE('',*,*,#3592,.T.);
#4706=ORIENTED_EDGE('',*,*,#3558,.T.);
#4707=ORIENTED_EDGE('',*,*,#3598,.T.);
#4708=ORIENTED_EDGE('',*,*,#3583,.F.);
#4709=ORIENTED_EDGE('',*,*,#3561,.T.);
#4710=ORIENTED_EDGE('',*,*,#3597,.T.);
#4711=ORIENTED_EDGE('',*,*,#3580,.F.);
#4712=ORIENTED_EDGE('',*,*,#3599,.F.);
#4713=ORIENTED_EDGE('',*,*,#3562,.T.);
#4714=ORIENTED_EDGE('',*,*,#3599,.T.);
#4715=ORIENTED_EDGE('',*,*,#3579,.F.);
#4716=ORIENTED_EDGE('',*,*,#3600,.F.);
#4717=ORIENTED_EDGE('',*,*,#3563,.T.);
#4718=ORIENTED_EDGE('',*,*,#3600,.T.);
#4719=ORIENTED_EDGE('',*,*,#3578,.F.);
#4720=ORIENTED_EDGE('',*,*,#3596,.F.);
#6601=CYLINDRICAL_SURFACE('',#7274,0.17);
#6602=CYLINDRICAL_SURFACE('',#7277,0.17);
#6603=CYLINDRICAL_SURFACE('',#7280,0.41);
#6604=CYLINDRICAL_SURFACE('',#7289,0.2);
#6605=CYLINDRICAL_SURFACE('',#7292,17.7082646568653);
#6606=CYLINDRICAL_SURFACE('',#7307,1.4);
#6607=CYLINDRICAL_SURFACE('',#7309,1.4);
#6608=CYLINDRICAL_SURFACE('',#7318,1.1);
#6609=CYLINDRICAL_SURFACE('',#7323,1.7);
#6610=CYLINDRICAL_SURFACE('',#7324,1.7);
#6742=ADVANCED_FACE('',(#820),#6601,.F.);
#6743=ADVANCED_FACE('',(#821),#6602,.F.);
#6744=ADVANCED_FACE('',(#822),#6603,.F.);
#6745=ADVANCED_FACE('',(#823),#653,.F.);
#6746=ADVANCED_FACE('',(#824),#654,.F.);
#6747=ADVANCED_FACE('',(#825),#655,.T.);
#6748=ADVANCED_FACE('',(#826),#656,.T.);
#6749=ADVANCED_FACE('',(#827),#657,.T.);
#6750=ADVANCED_FACE('',(#828),#6604,.T.);
#6751=ADVANCED_FACE('',(#829),#6605,.T.);
#6752=ADVANCED_FACE('',(#830),#658,.F.);
#6753=ADVANCED_FACE('',(#831),#659,.T.);
#6754=ADVANCED_FACE('',(#832),#660,.T.);
#6755=ADVANCED_FACE('',(#833),#661,.T.);
#6756=ADVANCED_FACE('',(#834),#662,.T.);
#6757=ADVANCED_FACE('',(#835),#663,.T.);
#6758=ADVANCED_FACE('',(#836,#582,#583,#584,#585),#664,.F.);
#6759=ADVANCED_FACE('',(#837),#665,.T.);
#6760=ADVANCED_FACE('',(#838),#6606,.T.);
#6761=ADVANCED_FACE('',(#839),#6607,.T.);
#6762=ADVANCED_FACE('',(#840,#586,#587,#588,#589),#666,.T.);
#6763=ADVANCED_FACE('',(#841),#578,.T.);
#6764=ADVANCED_FACE('',(#842),#6608,.F.);
#6765=ADVANCED_FACE('',(#843),#579,.T.);
#6766=ADVANCED_FACE('',(#844),#6609,.T.);
#6767=ADVANCED_FACE('',(#845),#6610,.T.);
#6768=ADVANCED_FACE('',(#846),#667,.T.);
#6769=ADVANCED_FACE('',(#847),#668,.T.);
#6770=ADVANCED_FACE('',(#848),#669,.T.);
#6771=ADVANCED_FACE('',(#849),#670,.T.);
#6772=ADVANCED_FACE('',(#850),#671,.T.);
#6773=ADVANCED_FACE('',(#851),#672,.T.);
#6774=ADVANCED_FACE('',(#852),#673,.T.);
#6775=ADVANCED_FACE('',(#853),#674,.T.);
#7151=CLOSED_SHELL('',(#6742,#6743,#6744,#6745,#6746,#6747,#6748,#6749,
#6750,#6751,#6752,#6753,#6754,#6755,#6756,#6757,#6758,#6759,#6760,#6761,
#6762,#6763,#6764,#6765,#6766,#6767,#6768,#6769,#6770,#6771,#6772,#6773,
#6774,#6775));
#7273=AXIS2_PLACEMENT_3D('',#9388,#7821,#7822);
#7274=AXIS2_PLACEMENT_3D('',#9389,#7823,#7824);
#7275=AXIS2_PLACEMENT_3D('',#9391,#7825,#7826);
#7276=AXIS2_PLACEMENT_3D('',#9394,#7828,#7829);
#7277=AXIS2_PLACEMENT_3D('',#9395,#7830,#7831);
#7278=AXIS2_PLACEMENT_3D('',#9397,#7832,#7833);
#7279=AXIS2_PLACEMENT_3D('',#9400,#7835,#7836);
#7280=AXIS2_PLACEMENT_3D('',#9401,#7837,#7838);
#7281=AXIS2_PLACEMENT_3D('',#9403,#7839,#7840);
#7282=AXIS2_PLACEMENT_3D('',#9406,#7842,#7843);
#7283=AXIS2_PLACEMENT_3D('',#9407,#7844,#7845);
#7284=AXIS2_PLACEMENT_3D('',#9414,#7849,#7850);
#7285=AXIS2_PLACEMENT_3D('',#9420,#7854,#7855);
#7286=AXIS2_PLACEMENT_3D('',#9424,#7858,#7859);
#7287=AXIS2_PLACEMENT_3D('',#9435,#7865,#7866);
#7288=AXIS2_PLACEMENT_3D('',#9436,#7867,#7868);
#7289=AXIS2_PLACEMENT_3D('',#9440,#7871,#7872);
#7290=AXIS2_PLACEMENT_3D('',#9442,#7873,#7874);
#7291=AXIS2_PLACEMENT_3D('',#9443,#7875,#7876);
#7292=AXIS2_PLACEMENT_3D('',#9445,#7878,#7879);
#7293=AXIS2_PLACEMENT_3D('',#9447,#7880,#7881);
#7294=AXIS2_PLACEMENT_3D('',#9449,#7883,#7884);
#7295=AXIS2_PLACEMENT_3D('',#9453,#7887,#7888);
#7296=AXIS2_PLACEMENT_3D('',#9459,#7892,#7893);
#7297=AXIS2_PLACEMENT_3D('',#9467,#7898,#7899);
#7298=AXIS2_PLACEMENT_3D('',#9471,#7902,#7903);
#7299=AXIS2_PLACEMENT_3D('',#9472,#7904,#7905);
#7300=AXIS2_PLACEMENT_3D('',#9478,#7909,#7910);
#7301=AXIS2_PLACEMENT_3D('',#9482,#7912,#7913);
#7302=AXIS2_PLACEMENT_3D('',#9488,#7916,#7917);
#7303=AXIS2_PLACEMENT_3D('',#9500,#7923,#7924);
#7304=AXIS2_PLACEMENT_3D('',#9503,#7926,#7927);
#7305=AXIS2_PLACEMENT_3D('',#9505,#7928,#7929);
#7306=AXIS2_PLACEMENT_3D('',#9506,#7930,#7931);
#7307=AXIS2_PLACEMENT_3D('',#9510,#7934,#7935);
#7308=AXIS2_PLACEMENT_3D('',#9513,#7937,#7938);
#7309=AXIS2_PLACEMENT_3D('',#9514,#7939,#7940);
#7310=AXIS2_PLACEMENT_3D('',#9516,#7941,#7942);
#7311=AXIS2_PLACEMENT_3D('',#9518,#7944,#7945);
#7312=AXIS2_PLACEMENT_3D('',#9522,#7947,#7948);
#7313=AXIS2_PLACEMENT_3D('',#9534,#7954,#7955);
#7314=AXIS2_PLACEMENT_3D('',#9539,#7958,#7959);
#7315=AXIS2_PLACEMENT_3D('',#9540,#7960,#7961);
#7316=AXIS2_PLACEMENT_3D('',#9542,#7962,#7963);
#7317=AXIS2_PLACEMENT_3D('',#9543,#7964,#7965);
#7318=AXIS2_PLACEMENT_3D('',#9544,#7966,#7967);
#7319=AXIS2_PLACEMENT_3D('',#9547,#7968,#7969);
#7320=AXIS2_PLACEMENT_3D('',#9548,#7970,#7971);
#7321=AXIS2_PLACEMENT_3D('',#9550,#7973,#7974);
#7322=AXIS2_PLACEMENT_3D('',#9551,#7975,#7976);
#7323=AXIS2_PLACEMENT_3D('',#9552,#7977,#7978);
#7324=AXIS2_PLACEMENT_3D('',#9555,#7981,#7982);
#7325=AXIS2_PLACEMENT_3D('',#9558,#7985,#7986);
#7326=AXIS2_PLACEMENT_3D('',#9560,#7988,#7989);
#7327=AXIS2_PLACEMENT_3D('',#9562,#7991,#7992);
#7328=AXIS2_PLACEMENT_3D('',#9563,#7993,#7994);
#7329=AXIS2_PLACEMENT_3D('',#9565,#7996,#7997);
#7330=AXIS2_PLACEMENT_3D('',#9566,#7998,#7999);
#7331=AXIS2_PLACEMENT_3D('',#9568,#8001,#8002);
#7332=AXIS2_PLACEMENT_3D('',#9570,#8004,#8005);
#7821=DIRECTION('axis',(0.,0.,1.));
#7822=DIRECTION('refdir',(1.,0.,0.));
#7823=DIRECTION('center_axis',(0.,0.,-1.));
#7824=DIRECTION('ref_axis',(1.,0.,0.));
#7825=DIRECTION('center_axis',(0.,0.,-1.));
#7826=DIRECTION('ref_axis',(1.,0.,0.));
#7827=DIRECTION('',(0.,0.,-1.));
#7828=DIRECTION('center_axis',(0.,0.,1.));
#7829=DIRECTION('ref_axis',(1.,0.,0.));
#7830=DIRECTION('center_axis',(0.,0.,-1.));
#7831=DIRECTION('ref_axis',(1.,0.,0.));
#7832=DIRECTION('center_axis',(0.,0.,-1.));
#7833=DIRECTION('ref_axis',(1.,0.,0.));
#7834=DIRECTION('',(0.,0.,-1.));
#7835=DIRECTION('center_axis',(0.,0.,1.));
#7836=DIRECTION('ref_axis',(1.,0.,0.));
#7837=DIRECTION('center_axis',(0.,0.,-1.));
#7838=DIRECTION('ref_axis',(1.,0.,0.));
#7839=DIRECTION('center_axis',(0.,0.,-1.));
#7840=DIRECTION('ref_axis',(1.,0.,0.));
#7841=DIRECTION('',(0.,0.,-1.));
#7842=DIRECTION('center_axis',(0.,0.,1.));
#7843=DIRECTION('ref_axis',(1.,0.,0.));
#7844=DIRECTION('center_axis',(1.,0.,0.));
#7845=DIRECTION('ref_axis',(0.,0.,-1.));
#7846=DIRECTION('',(0.,-1.,0.));
#7847=DIRECTION('',(0.,0.8,0.6));
#7848=DIRECTION('',(0.,0.,1.));
#7849=DIRECTION('center_axis',(0.,0.6,-0.8));
#7850=DIRECTION('ref_axis',(0.,0.8,0.6));
#7851=DIRECTION('',(0.,0.8,0.6));
#7852=DIRECTION('',(-1.,0.,0.));
#7853=DIRECTION('',(1.,0.,0.));
#7854=DIRECTION('center_axis',(1.,0.,0.));
#7855=DIRECTION('ref_axis',(0.,2.22044604925031E-16,1.));
#7856=DIRECTION('',(0.,1.,0.));
#7857=DIRECTION('',(0.,0.,1.));
#7858=DIRECTION('center_axis',(0.,0.,1.));
#7859=DIRECTION('ref_axis',(1.,0.,0.));
#7860=DIRECTION('',(0.6,0.8,0.));
#7861=DIRECTION('',(0.,-1.,0.));
#7862=DIRECTION('',(1.,0.,0.));
#7863=DIRECTION('',(0.,1.,0.));
#7864=DIRECTION('',(-1.,0.,0.));
#7865=DIRECTION('center_axis',(0.,0.,1.));
#7866=DIRECTION('ref_axis',(-0.0955793180441842,0.995421817101779,0.));
#7867=DIRECTION('center_axis',(0.8,-0.6,0.));
#7868=DIRECTION('ref_axis',(0.6,0.8,0.));
#7869=DIRECTION('',(0.,0.,-1.));
#7870=DIRECTION('',(-0.6,-0.8,0.));
#7871=DIRECTION('center_axis',(0.,0.,1.));
#7872=DIRECTION('ref_axis',(4.44089209850063E-15,1.,0.));
#7873=DIRECTION('center_axis',(0.,0.,1.));
#7874=DIRECTION('ref_axis',(4.44089209850063E-15,1.,0.));
#7875=DIRECTION('center_axis',(0.,0.,1.));
#7876=DIRECTION('ref_axis',(4.44089209850063E-15,1.,0.));
#7877=DIRECTION('',(0.,0.,1.));
#7878=DIRECTION('center_axis',(0.,0.,1.));
#7879=DIRECTION('ref_axis',(-0.0955793180441842,0.995421817101779,0.));
#7880=DIRECTION('center_axis',(0.,0.,1.));
#7881=DIRECTION('ref_axis',(-0.0955793180441842,0.995421817101779,0.));
#7882=DIRECTION('',(0.,0.,1.));
#7883=DIRECTION('center_axis',(0.,0.,1.));
#7884=DIRECTION('ref_axis',(1.,0.,0.));
#7885=DIRECTION('',(0.,1.,0.));
#7886=DIRECTION('',(1.,0.,0.));
#7887=DIRECTION('center_axis',(-1.,0.,0.));
#7888=DIRECTION('ref_axis',(0.,-1.,0.));
#7889=DIRECTION('',(0.,0.,1.));
#7890=DIRECTION('',(0.,1.,0.));
#7891=DIRECTION('',(0.,0.,1.));
#7892=DIRECTION('center_axis',(0.,1.,0.));
#7893=DIRECTION('ref_axis',(-1.,0.,0.));
#7894=DIRECTION('',(0.,0.,1.));
#7895=DIRECTION('',(-1.,0.,0.));
#7896=DIRECTION('',(0.,0.,1.));
#7897=DIRECTION('',(1.,0.,0.));
#7898=DIRECTION('center_axis',(1.,0.,0.));
#7899=DIRECTION('ref_axis',(0.,1.,0.));
#7900=DIRECTION('',(0.,0.,1.));
#7901=DIRECTION('',(0.,-1.,0.));
#7902=DIRECTION('center_axis',(0.,0.,1.));
#7903=DIRECTION('ref_axis',(1.,0.,0.));
#7904=DIRECTION('center_axis',(0.,-1.,0.));
#7905=DIRECTION('ref_axis',(1.,0.,0.));
#7906=DIRECTION('',(-1.,0.,0.));
#7907=DIRECTION('',(0.,0.,-1.));
#7908=DIRECTION('',(1.,0.,0.));
#7909=DIRECTION('center_axis',(0.,0.,1.));
#7910=DIRECTION('ref_axis',(1.,0.,0.));
#7911=DIRECTION('',(0.,-1.,0.));
#7912=DIRECTION('center_axis',(0.,0.,1.));
#7913=DIRECTION('ref_axis',(1.,0.,0.));
#7914=DIRECTION('',(-0.447213595499958,-0.894427190999916,0.));
#7915=DIRECTION('',(-0.694594513699567,0.719401460617409,0.));
#7916=DIRECTION('center_axis',(0.,0.,1.));
#7917=DIRECTION('ref_axis',(1.,0.,0.));
#7918=DIRECTION('',(-0.694594513699567,0.719401460617409,0.));
#7919=DIRECTION('',(-1.,0.,0.));
#7920=DIRECTION('',(0.,1.,0.));
#7921=DIRECTION('',(1.,0.,0.));
#7922=DIRECTION('',(0.87524153543927,-0.483686111690123,0.));
#7923=DIRECTION('center_axis',(0.,0.,1.));
#7924=DIRECTION('ref_axis',(1.,0.,0.));
#7925=DIRECTION('',(0.87524153543927,-0.483686111690123,0.));
#7926=DIRECTION('center_axis',(0.,0.,1.));
#7927=DIRECTION('ref_axis',(1.,0.,0.));
#7928=DIRECTION('center_axis',(0.,0.,-1.));
#7929=DIRECTION('ref_axis',(-1.,2.01858731750028E-16,0.));
#7930=DIRECTION('center_axis',(1.,0.,0.));
#7931=DIRECTION('ref_axis',(0.,1.,0.));
#7932=DIRECTION('',(0.,0.,1.));
#7933=DIRECTION('',(0.,1.,0.));
#7934=DIRECTION('center_axis',(0.,0.,1.));
#7935=DIRECTION('ref_axis',(1.,0.,0.));
#7936=DIRECTION('',(0.,0.,1.));
#7937=DIRECTION('center_axis',(0.,0.,1.));
#7938=DIRECTION('ref_axis',(1.,0.,0.));
#7939=DIRECTION('center_axis',(0.,0.,1.));
#7940=DIRECTION('ref_axis',(1.,0.,0.));
#7941=DIRECTION('center_axis',(0.,0.,1.));
#7942=DIRECTION('ref_axis',(1.,0.,0.));
#7943=DIRECTION('',(0.,0.,-1.));
#7944=DIRECTION('center_axis',(0.,0.,1.));
#7945=DIRECTION('ref_axis',(1.,0.,0.));
#7946=DIRECTION('',(0.87524153543927,-0.483686111690123,0.));
#7947=DIRECTION('center_axis',(0.,0.,1.));
#7948=DIRECTION('ref_axis',(1.,0.,0.));
#7949=DIRECTION('',(0.87524153543927,-0.483686111690123,0.));
#7950=DIRECTION('',(1.,0.,0.));
#7951=DIRECTION('',(0.,1.,0.));
#7952=DIRECTION('',(-1.,0.,0.));
#7953=DIRECTION('',(-0.694594513699567,0.719401460617409,0.));
#7954=DIRECTION('center_axis',(0.,0.,1.));
#7955=DIRECTION('ref_axis',(1.,0.,0.));
#7956=DIRECTION('',(-0.694594513699567,0.719401460617409,0.));
#7957=DIRECTION('',(-0.447213595499958,-0.894427190999916,0.));
#7958=DIRECTION('center_axis',(0.,0.,1.));
#7959=DIRECTION('ref_axis',(-1.,0.,0.));
#7960=DIRECTION('center_axis',(0.,0.,1.));
#7961=DIRECTION('ref_axis',(1.,0.,0.));
#7962=DIRECTION('center_axis',(0.,-1.,0.));
#7963=DIRECTION('ref_axis',(-1.,0.,0.));
#7964=DIRECTION('center_axis',(0.,0.,1.));
#7965=DIRECTION('ref_axis',(-1.,2.01858731750028E-16,0.));
#7966=DIRECTION('center_axis',(0.,0.,-1.));
#7967=DIRECTION('ref_axis',(1.,0.,0.));
#7968=DIRECTION('center_axis',(0.,0.,-1.));
#7969=DIRECTION('ref_axis',(-1.,0.,0.));
#7970=DIRECTION('center_axis',(0.,0.,-1.));
#7971=DIRECTION('ref_axis',(-1.,0.,0.));
#7972=DIRECTION('',(0.,0.,-1.));
#7973=DIRECTION('center_axis',(0.,0.,-1.));
#7974=DIRECTION('ref_axis',(-1.,0.,0.));
#7975=DIRECTION('center_axis',(0.,-1.,0.));
#7976=DIRECTION('ref_axis',(1.,0.,0.));
#7977=DIRECTION('center_axis',(0.,0.,1.));
#7978=DIRECTION('ref_axis',(1.,0.,0.));
#7979=DIRECTION('',(0.,0.,-1.));
#7980=DIRECTION('',(0.,0.,1.));
#7981=DIRECTION('center_axis',(0.,0.,1.));
#7982=DIRECTION('ref_axis',(-0.483686111690122,-0.87524153543927,0.));
#7983=DIRECTION('',(0.,0.,1.));
#7984=DIRECTION('',(0.,0.,-1.));
#7985=DIRECTION('center_axis',(-0.483686111690123,-0.87524153543927,0.));
#7986=DIRECTION('ref_axis',(0.87524153543927,-0.483686111690123,0.));
#7987=DIRECTION('',(0.,0.,1.));
#7988=DIRECTION('center_axis',(0.719401460617409,0.694594513699567,0.));
#7989=DIRECTION('ref_axis',(-0.694594513699567,0.719401460617409,0.));
#7990=DIRECTION('',(0.,0.,1.));
#7991=DIRECTION('center_axis',(-0.483686111690123,-0.87524153543927,0.));
#7992=DIRECTION('ref_axis',(0.87524153543927,-0.483686111690123,0.));
#7993=DIRECTION('center_axis',(-0.894427190999916,0.447213595499958,0.));
#7994=DIRECTION('ref_axis',(-0.447213595499958,-0.894427190999916,0.));
#7995=DIRECTION('',(0.,0.,1.));
#7996=DIRECTION('center_axis',(0.719401460617409,0.694594513699567,0.));
#7997=DIRECTION('ref_axis',(-0.694594513699567,0.719401460617409,0.));
#7998=DIRECTION('center_axis',(0.,1.,0.));
#7999=DIRECTION('ref_axis',(-1.,0.,0.));
#8000=DIRECTION('',(0.,0.,1.));
#8001=DIRECTION('center_axis',(1.,0.,0.));
#8002=DIRECTION('ref_axis',(0.,1.,0.));
#8003=DIRECTION('',(0.,0.,1.));
#8004=DIRECTION('center_axis',(0.,-1.,0.));
#8005=DIRECTION('ref_axis',(1.,0.,0.));
#9388=CARTESIAN_POINT('',(0.,0.,0.));
#9389=CARTESIAN_POINT('Origin',(6.,-2.5,0.3));
#9390=CARTESIAN_POINT('',(5.83,-2.5,0.6));
#9391=CARTESIAN_POINT('Origin',(6.,-2.5,0.6));
#9392=CARTESIAN_POINT('',(5.83,-2.5,0.));
#9393=CARTESIAN_POINT('',(5.83,-2.5,0.3));
#9394=CARTESIAN_POINT('Origin',(6.,-2.5,0.));
#9395=CARTESIAN_POINT('Origin',(14.,-2.5,0.3));
#9396=CARTESIAN_POINT('',(13.83,-2.5,0.6));
#9397=CARTESIAN_POINT('Origin',(14.,-2.5,0.6));
#9398=CARTESIAN_POINT('',(13.83,-2.5,0.));
#9399=CARTESIAN_POINT('',(13.83,-2.5,0.3));
#9400=CARTESIAN_POINT('Origin',(14.,-2.5,0.));
#9401=CARTESIAN_POINT('Origin',(0.,0.,0.3));
#9402=CARTESIAN_POINT('',(-0.41,5.02105187650415E-17,0.6));
#9403=CARTESIAN_POINT('Origin',(0.,0.,0.6));
#9404=CARTESIAN_POINT('',(-0.41,5.02105187650415E-17,0.));
#9405=CARTESIAN_POINT('',(-0.41,5.02105187650415E-17,0.3));
#9406=CARTESIAN_POINT('Origin',(0.,0.,0.));
#9407=CARTESIAN_POINT('Origin',(-2.2,-0.025,0.975));
#9408=CARTESIAN_POINT('',(-2.2,0.2,1.1));
#9409=CARTESIAN_POINT('',(-2.2,-0.2,1.1));
#9410=CARTESIAN_POINT('',(-2.2,0.2875,1.1));
#9411=CARTESIAN_POINT('',(-2.2,-0.2,0.8));
#9412=CARTESIAN_POINT('',(-2.2,-0.2,0.8));
#9413=CARTESIAN_POINT('',(-2.2,-0.2,0.8));
#9414=CARTESIAN_POINT('Origin',(-6.8,-0.2,0.8));
#9415=CARTESIAN_POINT('',(-6.8,-0.2,0.8));
#9416=CARTESIAN_POINT('',(-6.8,0.199999999999998,1.1));
#9417=CARTESIAN_POINT('',(-6.8,-0.2,0.8));
#9418=CARTESIAN_POINT('',(-2.2,-0.2,0.8));
#9419=CARTESIAN_POINT('',(-4.3,0.2,1.1));
#9420=CARTESIAN_POINT('Origin',(-6.8,-0.025,0.975));
#9421=CARTESIAN_POINT('',(-6.8,-0.2,1.1));
#9422=CARTESIAN_POINT('',(-6.8,0.2875,1.1));
#9423=CARTESIAN_POINT('',(-6.8,-0.2,0.8));
#9424=CARTESIAN_POINT('Origin',(-1.8,0.6,1.1));
#9425=CARTESIAN_POINT('',(-2.,0.0666666666666668,1.1));
#9426=CARTESIAN_POINT('',(-1.6,0.6,1.1));
#9427=CARTESIAN_POINT('',(-2.,0.,1.1));
#9428=CARTESIAN_POINT('',(-2.,0.,1.1));
#9429=CARTESIAN_POINT('',(-1.6,0.,1.1));
#9430=CARTESIAN_POINT('',(-1.6,0.,1.1));
#9431=CARTESIAN_POINT('',(-1.6,1.2,1.1));
#9432=CARTESIAN_POINT('',(-1.6,1.2,1.1));
#9433=CARTESIAN_POINT('',(-2.4,1.2,1.1));
#9434=CARTESIAN_POINT('',(-2.,1.2,1.1));
#9435=CARTESIAN_POINT('Origin',(-0.70745614035088,-16.4271929824561,1.1));
#9436=CARTESIAN_POINT('Origin',(-2.2,-0.2,0.8));
#9437=CARTESIAN_POINT('',(-2.,0.0666666666666669,0.8));
#9438=CARTESIAN_POINT('',(-2.,0.0666666666666667,0.4));
#9439=CARTESIAN_POINT('',(-1.6,0.6,0.8));
#9440=CARTESIAN_POINT('Origin',(-6.8,1.38777878078145E-17,0.8));
#9441=CARTESIAN_POINT('',(-6.8,0.199999999999998,0.8));
#9442=CARTESIAN_POINT('Origin',(-6.8,1.38777878078145E-17,0.8));
#9443=CARTESIAN_POINT('Origin',(-6.8,1.38777878078145E-17,1.1));
#9444=CARTESIAN_POINT('',(-6.8,0.199999999999998,0.8));
#9445=CARTESIAN_POINT('Origin',(-0.70745614035088,-16.4271929824561,0.8));
#9446=CARTESIAN_POINT('',(-2.4,1.2,0.8));
#9447=CARTESIAN_POINT('Origin',(-0.70745614035088,-16.4271929824561,0.8));
#9448=CARTESIAN_POINT('',(-2.4,1.2,0.8));
#9449=CARTESIAN_POINT('Origin',(-4.3,0.5,0.8));
#9450=CARTESIAN_POINT('',(-2.,1.2,0.8));
#9451=CARTESIAN_POINT('',(-2.,0.85,0.8));
#9452=CARTESIAN_POINT('',(-2.4,1.2,0.8));
#9453=CARTESIAN_POINT('Origin',(-2.,1.2,0.));
#9454=CARTESIAN_POINT('',(-2.,1.2,0.));
#9455=CARTESIAN_POINT('',(-2.,1.2,0.));
#9456=CARTESIAN_POINT('',(-2.,0.,0.));
#9457=CARTESIAN_POINT('',(-2.,0.,0.));
#9458=CARTESIAN_POINT('',(-2.,0.,0.));
#9459=CARTESIAN_POINT('Origin',(-1.2,1.2,0.));
#9460=CARTESIAN_POINT('',(-1.6,1.2,0.6));
#9461=CARTESIAN_POINT('',(-1.6,1.2,0.));
#9462=CARTESIAN_POINT('',(-1.2,1.2,0.6));
#9463=CARTESIAN_POINT('',(-2.,1.2,0.6));
#9464=CARTESIAN_POINT('',(-1.2,1.2,0.));
#9465=CARTESIAN_POINT('',(-1.2,1.2,0.));
#9466=CARTESIAN_POINT('',(-2.,1.2,0.));
#9467=CARTESIAN_POINT('Origin',(-1.6,0.,0.));
#9468=CARTESIAN_POINT('',(-1.6,0.,0.6));
#9469=CARTESIAN_POINT('',(-1.6,0.,0.));
#9470=CARTESIAN_POINT('',(-1.6,0.,0.6));
#9471=CARTESIAN_POINT('Origin',(-1.8,0.6,1.1));
#9472=CARTESIAN_POINT('Origin',(-2.,0.,0.));
#9473=CARTESIAN_POINT('',(-1.4,0.,0.));
#9474=CARTESIAN_POINT('',(-1.2,0.,0.));
#9475=CARTESIAN_POINT('',(-1.4,0.,0.6));
#9476=CARTESIAN_POINT('',(-1.4,0.,0.));
#9477=CARTESIAN_POINT('',(-1.2,0.,0.6));
#9478=CARTESIAN_POINT('Origin',(0.,0.,0.));
#9479=CARTESIAN_POINT('',(-1.2,0.721110255092798,0.));
#9480=CARTESIAN_POINT('',(-1.2,1.2,0.));
#9481=CARTESIAN_POINT('',(0.993295878967653,0.986591757935306,0.));
#9482=CARTESIAN_POINT('Origin',(0.,0.,0.));
#9483=CARTESIAN_POINT('',(1.,1.,0.));
#9484=CARTESIAN_POINT('',(1.,1.,0.));
#9485=CARTESIAN_POINT('',(2.26270761578574,-0.307804316349519,0.));
#9486=CARTESIAN_POINT('',(3.8,-1.9,0.));
#9487=CARTESIAN_POINT('',(3.79686161498349,-1.89674952980433,0.));
#9488=CARTESIAN_POINT('Origin',(2.1,-2.,0.));
#9489=CARTESIAN_POINT('',(3.8,-1.9,0.));
#9490=CARTESIAN_POINT('',(3.8,-1.9,0.));
#9491=CARTESIAN_POINT('',(15.2,-1.9,0.));
#9492=CARTESIAN_POINT('',(15.2,-1.9,0.));
#9493=CARTESIAN_POINT('',(15.2,-3.1,0.));
#9494=CARTESIAN_POINT('',(15.2,-3.1,0.));
#9495=CARTESIAN_POINT('',(3.8,-3.1,0.));
#9496=CARTESIAN_POINT('',(3.8,-3.1,0.));
#9497=CARTESIAN_POINT('',(3.51486278039743,-2.94242416811437,0.));
#9498=CARTESIAN_POINT('',(0.,-1.,0.));
#9499=CARTESIAN_POINT('',(0.549222100239177,-1.30351747644797,0.));
#9500=CARTESIAN_POINT('Origin',(2.1,-2.,0.));
#9501=CARTESIAN_POINT('',(0.533017816115691,-1.29456247732709,0.));
#9502=CARTESIAN_POINT('',(0.,-1.,0.));
#9503=CARTESIAN_POINT('Origin',(0.,0.,0.));
#9504=CARTESIAN_POINT('',(0.9,-2.,0.));
#9505=CARTESIAN_POINT('Origin',(2.1,-2.,0.));
#9506=CARTESIAN_POINT('Origin',(-1.2,0.,0.));
#9507=CARTESIAN_POINT('',(-1.2,0.721110255092798,0.6));
#9508=CARTESIAN_POINT('',(-1.2,0.721110255092798,0.));
#9509=CARTESIAN_POINT('',(-1.2,1.2,0.6));
#9510=CARTESIAN_POINT('Origin',(0.,0.,0.));
#9511=CARTESIAN_POINT('',(0.533017816115691,-1.29456247732709,0.6));
#9512=CARTESIAN_POINT('',(0.533017816115691,-1.29456247732709,0.));
#9513=CARTESIAN_POINT('Origin',(0.,0.,0.6));
#9514=CARTESIAN_POINT('Origin',(0.,0.,0.));
#9515=CARTESIAN_POINT('',(0.993295878967653,0.986591757935306,0.6));
#9516=CARTESIAN_POINT('Origin',(0.,0.,0.6));
#9517=CARTESIAN_POINT('',(0.993295878967653,0.986591757935306,0.));
#9518=CARTESIAN_POINT('Origin',(0.,0.,0.6));
#9519=CARTESIAN_POINT('',(0.549222100239177,-1.30351747644797,0.6));
#9520=CARTESIAN_POINT('',(0.,-1.,0.6));
#9521=CARTESIAN_POINT('',(3.51486278039743,-2.94242416811437,0.6));
#9522=CARTESIAN_POINT('Origin',(2.1,-2.,0.6));
#9523=CARTESIAN_POINT('',(3.8,-3.1,0.6));
#9524=CARTESIAN_POINT('',(0.,-1.,0.6));
#9525=CARTESIAN_POINT('',(15.2,-3.1,0.6));
#9526=CARTESIAN_POINT('',(3.8,-3.1,0.6));
#9527=CARTESIAN_POINT('',(15.2,-1.9,0.6));
#9528=CARTESIAN_POINT('',(15.2,-3.1,0.6));
#9529=CARTESIAN_POINT('',(3.8,-1.9,0.6));
#9530=CARTESIAN_POINT('',(15.2,-1.9,0.6));
#9531=CARTESIAN_POINT('',(3.79686161498349,-1.89674952980433,0.6));
#9532=CARTESIAN_POINT('',(3.8,-1.9,0.6));
#9533=CARTESIAN_POINT('',(2.26270761578574,-0.307804316349519,0.6));
#9534=CARTESIAN_POINT('Origin',(2.1,-2.,0.6));
#9535=CARTESIAN_POINT('',(1.,1.,0.6));
#9536=CARTESIAN_POINT('',(3.8,-1.9,0.6));
#9537=CARTESIAN_POINT('',(1.,1.,0.6));
#9538=CARTESIAN_POINT('',(3.3,-2.,0.6));
#9539=CARTESIAN_POINT('Origin',(2.1,-2.,0.6));
#9540=CARTESIAN_POINT('Origin',(2.1,-2.,0.1));
#9541=CARTESIAN_POINT('',(1.,-2.,0.1));
#9542=CARTESIAN_POINT('Origin',(0.9,-2.,0.1));
#9543=CARTESIAN_POINT('Origin',(2.1,-2.,0.1));
#9544=CARTESIAN_POINT('Origin',(2.1,-2.,0.3));
#9545=CARTESIAN_POINT('',(3.2,-2.,0.5));
#9546=CARTESIAN_POINT('',(1.,-2.,0.5));
#9547=CARTESIAN_POINT('Origin',(2.1,-2.,0.5));
#9548=CARTESIAN_POINT('Origin',(2.1,-2.,0.5));
#9549=CARTESIAN_POINT('',(1.,-2.,0.3));
#9550=CARTESIAN_POINT('Origin',(2.1,-2.,0.5));
#9551=CARTESIAN_POINT('Origin',(3.3,-2.,0.5));
#9552=CARTESIAN_POINT('Origin',(2.1,-2.,0.));
#9553=CARTESIAN_POINT('',(2.26270761578574,-0.307804316349519,0.));
#9554=CARTESIAN_POINT('',(3.79686161498349,-1.89674952980433,0.));
#9555=CARTESIAN_POINT('Origin',(2.1,-2.,0.));
#9556=CARTESIAN_POINT('',(0.549222100239177,-1.30351747644797,0.));
#9557=CARTESIAN_POINT('',(3.51486278039743,-2.94242416811437,0.));
#9558=CARTESIAN_POINT('Origin',(0.,-1.,0.));
#9559=CARTESIAN_POINT('',(3.8,-3.1,0.));
#9560=CARTESIAN_POINT('Origin',(3.8,-1.9,0.));
#9561=CARTESIAN_POINT('',(3.8,-1.9,0.));
#9562=CARTESIAN_POINT('Origin',(0.,-1.,0.));
#9563=CARTESIAN_POINT('Origin',(1.,1.,0.));
#9564=CARTESIAN_POINT('',(1.,1.,0.));
#9565=CARTESIAN_POINT('Origin',(3.8,-1.9,0.));
#9566=CARTESIAN_POINT('Origin',(15.2,-1.9,0.));
#9567=CARTESIAN_POINT('',(15.2,-1.9,0.));
#9568=CARTESIAN_POINT('Origin',(15.2,-3.1,0.));
#9569=CARTESIAN_POINT('',(15.2,-3.1,0.));
#9570=CARTESIAN_POINT('Origin',(3.8,-3.1,0.));
#19447=UNCERTAINTY_MEASURE_WITH_UNIT(LENGTH_MEASURE(0.001),#19472,
'DISTANCE_ACCURACY_VALUE',
'Maximum model space distance between geometric entities at asserted c
onnectivities');
#19458=UNCERTAINTY_MEASURE_WITH_UNIT(LENGTH_MEASURE(0.001),#19472,
'DISTANCE_ACCURACY_VALUE',
'Maximum model space distance between geometric entities at asserted c
onnectivities');
#19460=(
GEOMETRIC_REPRESENTATION_CONTEXT(3)
GLOBAL_UNCERTAINTY_ASSIGNED_CONTEXT((#19447))
GLOBAL_UNIT_ASSIGNED_CONTEXT((#19472,#19474,#19475))
REPRESENTATION_CONTEXT('','3D')
);
#19471=(
GEOMETRIC_REPRESENTATION_CONTEXT(3)
GLOBAL_UNCERTAINTY_ASSIGNED_CONTEXT((#19458))
GLOBAL_UNIT_ASSIGNED_CONTEXT((#19472,#19474,#19475))
REPRESENTATION_CONTEXT('','3D')
);
#19472=(
LENGTH_UNIT()
NAMED_UNIT(*)
SI_UNIT(.CENTI.,.METRE.)
);
#19474=(
NAMED_UNIT(*)
PLANE_ANGLE_UNIT()
SI_UNIT($,.RADIAN.)
);
#19475=(
NAMED_UNIT(*)
SI_UNIT($,.STERADIAN.)
SOLID_ANGLE_UNIT()
);
#19477=SHAPE_DEFINITION_REPRESENTATION(#19489,#19517);
#19489=PRODUCT_DEFINITION_SHAPE('',$,#19530);
#19517=SHAPE_REPRESENTATION('',(#7273),#19460);
#19528=PRODUCT_DEFINITION_CONTEXT('part definition',#19566,'design');
#19530=PRODUCT_DEFINITION('Forged jaw and handle',
'Forged jaw and handle',#19542,#19528);
#19542=PRODUCT_DEFINITION_FORMATION('',$,#19569);
#19566=APPLICATION_CONTEXT(
'Core Data for Automotive Mechanical Design Process');
#19567=PRODUCT_CONTEXT('part definition',#19566,'mechanical');
#19569=PRODUCT('Forged jaw and handle','Forged jaw and handle',$,(#19567));
#19581=PRESENTATION_STYLE_ASSIGNMENT((#19589));
#19589=SURFACE_STYLE_USAGE(.BOTH.,#19597);
#19597=SURFACE_SIDE_STYLE('',(#19605));
#19605=SURFACE_STYLE_FILL_AREA(#19613);
#19613=FILL_AREA_STYLE('Tool steel gray',(#19621));
#19621=FILL_AREA_STYLE_COLOUR('Tool steel gray',#19629);
#19629=COLOUR_RGB('Tool steel gray',0.607843137254902,0.643137254901961,
0.698039215686274);
ENDSEC;
END-ISO-10303-21;
